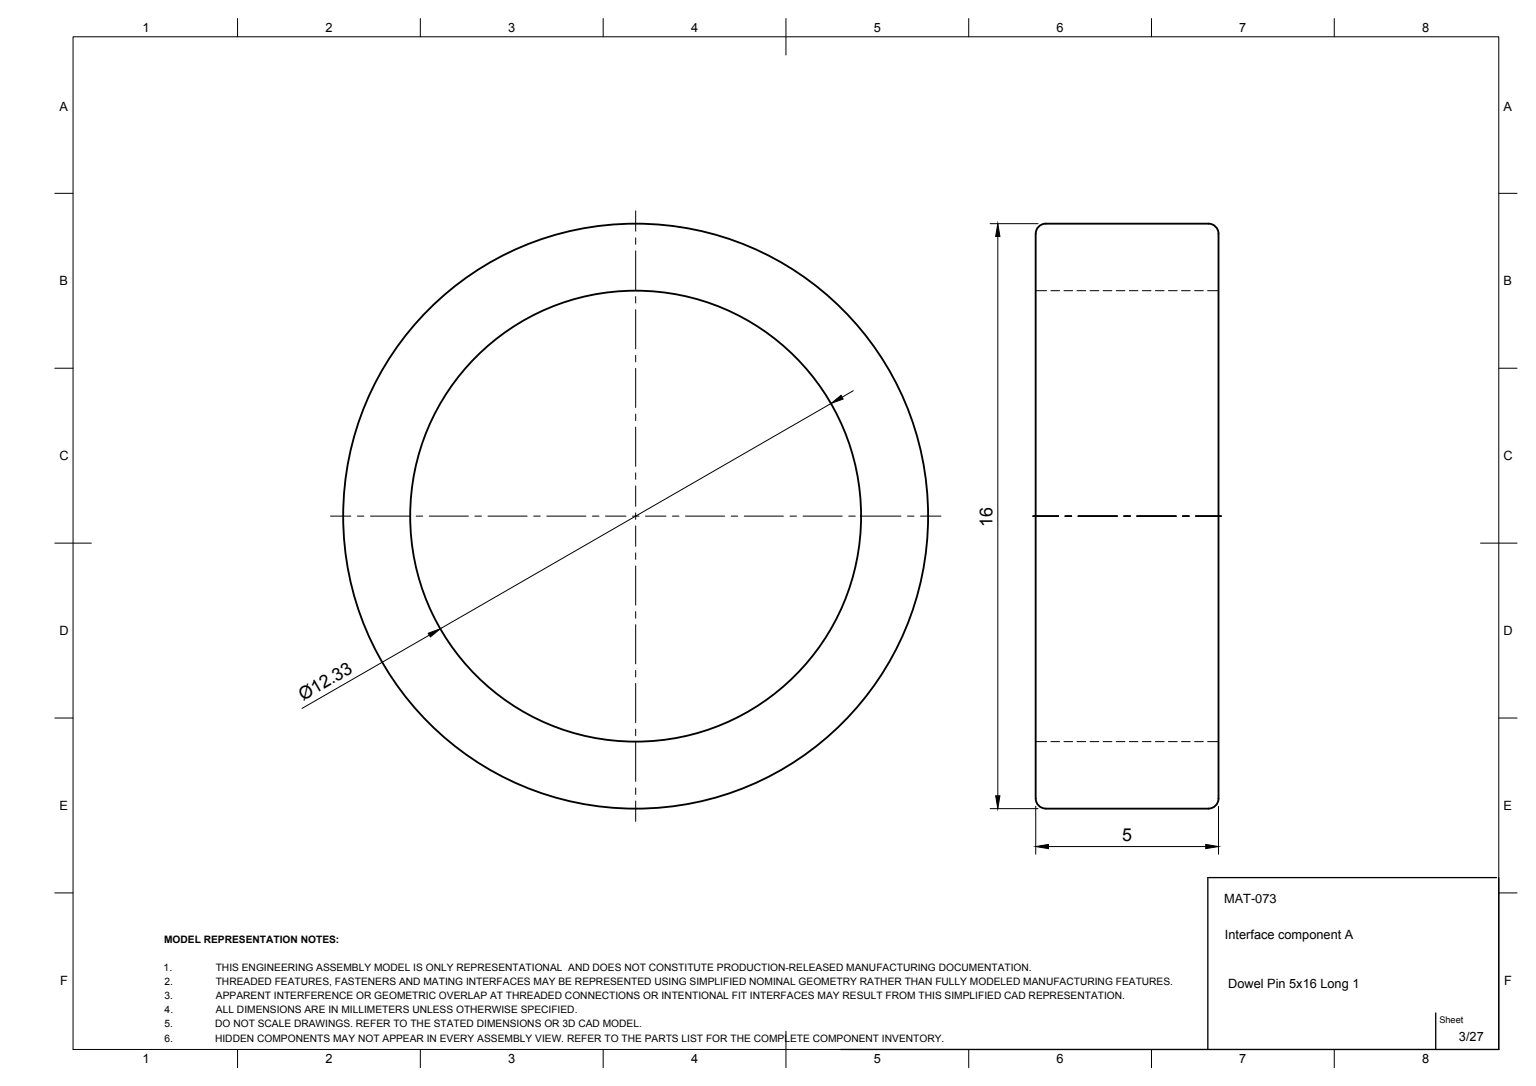
ISO-10303-21;
HEADER;
/* Generated by software containing ST-Developer
 * from STEP Tools, Inc. (www.steptools.com) 
 */

FILE_DESCRIPTION(
/* description */ ('CAx-IF Rec.Pracs.---Representation and Presentation of Product Manufa
cturing Information (PMI)---4.0---2014-10-13'),
/* implementation_level */ '2;1');

FILE_NAME(
/* name */ 'Interface component A.step',
/* time_stamp */ '2026-10-24T18:52:33-07:00',
/* author */ (''),
/* organization */ (''),
/* preprocessor_version */ 'ST-DEVELOPER v20.2',
/* originating_system */ 'Autodesk Translation Framework v15.17.0.0',
/* authorisation */ '');

FILE_SCHEMA (('AP242_MANAGED_MODEL_BASED_3D_ENGINEERING_MIM_LF { 1 0 10303 442 2 1 4 }'));
ENDSEC;

DATA;
#10=MECHANICAL_DESIGN_GEOMETRIC_PRESENTATION_REPRESENTATION('',(#414),#34876);
#348=SHAPE_REPRESENTATION_RELATIONSHIP('SRR','None',#34985,#381);
#381=ADVANCED_BREP_SHAPE_REPRESENTATION('',(#447),#34843);
#414=STYLED_ITEM('',(#35159),#447);
#447=MANIFOLD_SOLID_BREP('Dowel Pin 5x16 Long 1',#19554);
#480=FACE_BOUND('',#5841,.T.);
#481=FACE_BOUND('',#5844,.T.);
#590=PLANE('',#19961);
#591=PLANE('',#19966);
#1083=LINE('',#28483,#2682);
#1084=LINE('',#28498,#2683);
#2682=VECTOR('',#22274,0.008);
#2683=VECTOR('',#22295,0.00616666666666666);
#4281=CYLINDRICAL_SURFACE('',#19958,0.008);
#4282=CYLINDRICAL_SURFACE('',#19968,0.00616666666666666);
#4793=FACE_OUTER_BOUND('',#5838,.T.);
#4794=FACE_OUTER_BOUND('',#5839,.T.);
#4795=FACE_OUTER_BOUND('',#5840,.T.);
#4796=FACE_OUTER_BOUND('',#5842,.T.);
#4797=FACE_OUTER_BOUND('',#5843,.T.);
#4798=FACE_OUTER_BOUND('',#5845,.T.);
#5838=EDGE_LOOP('',(#12806,#12807,#12808,#12809,#12810));
#5839=EDGE_LOOP('',(#12811,#12812,#12813,#12814,#12815,#12816));
#5840=EDGE_LOOP('',(#12817));
#5841=EDGE_LOOP('',(#12818));
#5842=EDGE_LOOP('',(#12819,#12820,#12821,#12822,#12823));
#5843=EDGE_LOOP('',(#12824));
#5844=EDGE_LOOP('',(#12825));
#5845=EDGE_LOOP('',(#12826,#12827,#12828,#12829));
#6993=CIRCLE('',#19954,0.00772500000001);
#6994=CIRCLE('',#19955,0.000275);
#6995=CIRCLE('',#19956,0.00800000000001);
#6996=CIRCLE('',#19957,0.00800000000001);
#6997=CIRCLE('',#19959,0.00800000000001);
#6998=CIRCLE('',#19960,0.00800000000001);
#6999=CIRCLE('',#19962,0.00616666666667666);
#7000=CIRCLE('',#19964,0.000275);
#7001=CIRCLE('',#19965,0.00772500000001);
#7002=CIRCLE('',#19967,0.00616666666667666);
#8073=VERTEX_POINT('',#28474);
#8074=VERTEX_POINT('',#28476);
#8075=VERTEX_POINT('',#28478);
#8076=VERTEX_POINT('',#28482);
#8077=VERTEX_POINT('',#28484);
#8078=VERTEX_POINT('',#28488);
#8079=VERTEX_POINT('',#28491);
#8080=VERTEX_POINT('',#28495);
#9961=EDGE_CURVE('',#8073,#8073,#6993,.T.);
#9962=EDGE_CURVE('',#8073,#8074,#6994,.T.);
#9963=EDGE_CURVE('',#8074,#8075,#6995,.T.);
#9964=EDGE_CURVE('',#8075,#8074,#6996,.T.);
#9965=EDGE_CURVE('',#8075,#8076,#1083,.T.);
#9966=EDGE_CURVE('',#8077,#8076,#6997,.T.);
#9967=EDGE_CURVE('',#8076,#8077,#6998,.T.);
#9968=EDGE_CURVE('',#8078,#8078,#6999,.T.);
#9969=EDGE_CURVE('',#8077,#8079,#7000,.T.);
#9970=EDGE_CURVE('',#8079,#8079,#7001,.T.);
#9971=EDGE_CURVE('',#8080,#8080,#7002,.T.);
#9972=EDGE_CURVE('',#8080,#8078,#1084,.T.);
#12806=ORIENTED_EDGE('',*,*,#9961,.T.);
#12807=ORIENTED_EDGE('',*,*,#9962,.T.);
#12808=ORIENTED_EDGE('',*,*,#9963,.T.);
#12809=ORIENTED_EDGE('',*,*,#9964,.T.);
#12810=ORIENTED_EDGE('',*,*,#9962,.F.);
#12811=ORIENTED_EDGE('',*,*,#9964,.F.);
#12812=ORIENTED_EDGE('',*,*,#9965,.T.);
#12813=ORIENTED_EDGE('',*,*,#9966,.F.);
#12814=ORIENTED_EDGE('',*,*,#9967,.F.);
#12815=ORIENTED_EDGE('',*,*,#9965,.F.);
#12816=ORIENTED_EDGE('',*,*,#9963,.F.);
#12817=ORIENTED_EDGE('',*,*,#9961,.F.);
#12818=ORIENTED_EDGE('',*,*,#9968,.F.);
#12819=ORIENTED_EDGE('',*,*,#9967,.T.);
#12820=ORIENTED_EDGE('',*,*,#9969,.T.);
#12821=ORIENTED_EDGE('',*,*,#9970,.T.);
#12822=ORIENTED_EDGE('',*,*,#9969,.F.);
#12823=ORIENTED_EDGE('',*,*,#9966,.T.);
#12824=ORIENTED_EDGE('',*,*,#9970,.F.);
#12825=ORIENTED_EDGE('',*,*,#9971,.T.);
#12826=ORIENTED_EDGE('',*,*,#9971,.F.);
#12827=ORIENTED_EDGE('',*,*,#9972,.T.);
#12828=ORIENTED_EDGE('',*,*,#9968,.T.);
#12829=ORIENTED_EDGE('',*,*,#9972,.F.);
#18496=TOROIDAL_SURFACE('',#19953,0.007725,0.000275);
#18497=TOROIDAL_SURFACE('',#19963,0.007725,0.000275);
#18509=ADVANCED_FACE('',(#4793),#18496,.T.);
#18510=ADVANCED_FACE('',(#4794),#4281,.T.);
#18511=ADVANCED_FACE('',(#4795,#480),#590,.T.);
#18512=ADVANCED_FACE('',(#4796),#18497,.T.);
#18513=ADVANCED_FACE('',(#4797,#481),#591,.T.);
#18514=ADVANCED_FACE('',(#4798),#4282,.F.);
#19554=CLOSED_SHELL('',(#18509,#18510,#18511,#18512,#18513,#18514));
#19952=AXIS2_PLACEMENT_3D('',#28472,#22260,#22261);
#19953=AXIS2_PLACEMENT_3D('',#28473,#22262,#22263);
#19954=AXIS2_PLACEMENT_3D('',#28475,#22264,#22265);
#19955=AXIS2_PLACEMENT_3D('',#28477,#22266,#22267);
#19956=AXIS2_PLACEMENT_3D('',#28479,#22268,#22269);
#19957=AXIS2_PLACEMENT_3D('',#28480,#22270,#22271);
#19958=AXIS2_PLACEMENT_3D('',#28481,#22272,#22273);
#19959=AXIS2_PLACEMENT_3D('',#28485,#22275,#22276);
#19960=AXIS2_PLACEMENT_3D('',#28486,#22277,#22278);
#19961=AXIS2_PLACEMENT_3D('',#28487,#22279,#22280);
#19962=AXIS2_PLACEMENT_3D('',#28489,#22281,#22282);
#19963=AXIS2_PLACEMENT_3D('',#28490,#22283,#22284);
#19964=AXIS2_PLACEMENT_3D('',#28492,#22285,#22286);
#19965=AXIS2_PLACEMENT_3D('',#28493,#22287,#22288);
#19966=AXIS2_PLACEMENT_3D('',#28494,#22289,#22290);
#19967=AXIS2_PLACEMENT_3D('',#28496,#22291,#22292);
#19968=AXIS2_PLACEMENT_3D('',#28497,#22293,#22294);
#22260=DIRECTION('axis',(0.,0.,1.));
#22261=DIRECTION('refdir',(1.,0.,0.));
#22262=DIRECTION('center_axis',(4.55032717710333E-17,-1.,1.51850909121962E-32));
#22263=DIRECTION('ref_axis',(-0.770184521566975,0.,0.637821136948792));
#22264=DIRECTION('center_axis',(-4.55032717710333E-17,1.,-1.51850909121962E-32));
#22265=DIRECTION('ref_axis',(0.637821136949789,2.90229485359357E-17,0.770184521566149));
#22266=DIRECTION('center_axis',(0.637821136948792,2.90229485358903E-17,
0.770184521566975));
#22267=DIRECTION('ref_axis',(0.770184521566975,0.,-0.637821136948792));
#22268=DIRECTION('center_axis',(4.55032717710333E-17,-1.,1.51850909121962E-32));
#22269=DIRECTION('ref_axis',(0.637821136949755,2.90229485359342E-17,0.770184521566178));
#22270=DIRECTION('center_axis',(4.55032717710333E-17,-1.,1.51850909121962E-32));
#22271=DIRECTION('ref_axis',(0.637821136949755,2.90229485359342E-17,0.770184521566178));
#22272=DIRECTION('center_axis',(4.55032717710333E-17,-1.,1.51850909121962E-32));
#22273=DIRECTION('ref_axis',(-0.637821136948792,-2.90229485358903E-17,-0.770184521566975));
#22274=DIRECTION('',(-4.55032717710333E-17,1.,-1.51850909121962E-32));
#22275=DIRECTION('center_axis',(-4.55032717710333E-17,1.,-1.51850909121962E-32));
#22276=DIRECTION('ref_axis',(0.637821136949755,2.90229485359342E-17,0.770184521566178));
#22277=DIRECTION('center_axis',(-4.55032717710333E-17,1.,-1.51850909121962E-32));
#22278=DIRECTION('ref_axis',(0.637821136949755,2.90229485359342E-17,0.770184521566178));
#22279=DIRECTION('center_axis',(4.55032717710333E-17,-1.,1.51850909121962E-32));
#22280=DIRECTION('ref_axis',(-0.637821136948792,-2.90229485358903E-17,-0.770184521566975));
#22281=DIRECTION('center_axis',(4.55032717710333E-17,-1.,1.51850909121962E-32));
#22282=DIRECTION('ref_axis',(-0.637821136948792,-2.90229485358904E-17,-0.770184521566975));
#22283=DIRECTION('center_axis',(4.55032717710333E-17,-1.,1.51850909121962E-32));
#22284=DIRECTION('ref_axis',(-0.770184521566975,-5.42101086242752E-17,0.637821136948792));
#22285=DIRECTION('center_axis',(0.637821136948792,2.90229485358903E-17,
0.770184521566975));
#22286=DIRECTION('ref_axis',(0.770184521566975,3.46944695195361E-17,-0.637821136948792));
#22287=DIRECTION('center_axis',(4.55032717710333E-17,-1.,1.51850909121962E-32));
#22288=DIRECTION('ref_axis',(0.637821136949789,2.90229485359357E-17,0.770184521566149));
#22289=DIRECTION('center_axis',(-4.55032717710333E-17,1.,-1.51850909121962E-32));
#22290=DIRECTION('ref_axis',(0.770184521566975,3.50459155987053E-17,-0.637821136948792));
#22291=DIRECTION('center_axis',(4.55032717710333E-17,-1.,1.51850909121962E-32));
#22292=DIRECTION('ref_axis',(-0.637821136948792,-2.90229485358904E-17,-0.770184521566975));
#22293=DIRECTION('center_axis',(4.55032717710333E-17,-1.,1.51850909121962E-32));
#22294=DIRECTION('ref_axis',(-0.637821136948792,-2.90229485358903E-17,-0.770184521566975));
#22295=DIRECTION('',(4.55032717710333E-17,-1.,1.51850909121962E-32));
#28472=CARTESIAN_POINT('',(0.,0.,0.));
#28473=CARTESIAN_POINT('Origin',(-4.50826289289608E-17,-0.006725,1.13636778952413E-32));
#28474=CARTESIAN_POINT('',(0.00594967542911254,-0.00700000000001,-0.00492716828293579));
#28475=CARTESIAN_POINT('Origin',(-4.50701155292233E-17,-0.00700000000001,
1.13678537952423E-32));
#28476=CARTESIAN_POINT('',(0.00616147617254346,-0.00672500000001,-0.00510256909559671));
#28477=CARTESIAN_POINT('Origin',(0.00594967542910484,-0.006725,-0.00492716828292942));
#28478=CARTESIAN_POINT('',(0.00510256909560437,-0.00672500000001,0.00616147617253713));
#28479=CARTESIAN_POINT('Origin',(-4.50826289289603E-17,-0.00672500000001,
1.13636778952415E-32));
#28480=CARTESIAN_POINT('Origin',(-4.50826289289603E-17,-0.00672500000001,
1.13636778952415E-32));
#28481=CARTESIAN_POINT('Origin',(-4.51838737086513E-17,-0.0045,1.13298910679617E-32));
#28482=CARTESIAN_POINT('',(0.00510256909560437,-0.00227500000001,0.00616147617253713));
#28483=CARTESIAN_POINT('',(0.00510256909559029,-0.0045,0.0061614761725358));
#28484=CARTESIAN_POINT('',(0.00616147617254346,-0.00227500000001001,-0.00510256909559671));
#28485=CARTESIAN_POINT('Origin',(-4.52851184883414E-17,-0.00227500000001001,
1.12961042406822E-32));
#28486=CARTESIAN_POINT('Origin',(-4.52851184883414E-17,-0.00227500000001001,
1.12961042406822E-32));
#28487=CARTESIAN_POINT('Origin',(-0.00451789972005399,-0.007,-0.00545547369443274));
#28488=CARTESIAN_POINT('',(0.0039332303445175,-0.00700000000001,0.00474947121632968));
#28489=CARTESIAN_POINT('Origin',(-4.50701155292233E-17,-0.00700000000001,
1.13678537952423E-32));
#28490=CARTESIAN_POINT('Origin',(-4.52851184883419E-17,-0.002275,1.1296104240682E-32));
#28491=CARTESIAN_POINT('',(0.00594967542911254,-0.00200000000001001,-0.00492716828293579));
#28492=CARTESIAN_POINT('Origin',(0.00594967542910484,-0.002275,-0.00492716828292942));
#28493=CARTESIAN_POINT('Origin',(-4.52976318880785E-17,-0.00200000000001001,
1.12919283406813E-32));
#28494=CARTESIAN_POINT('Origin',(-0.00451789972005399,-0.002,-0.00545547369443274));
#28495=CARTESIAN_POINT('',(0.0039332303445175,-0.00200000000001001,0.00474947121632968));
#28496=CARTESIAN_POINT('Origin',(-4.52976318880785E-17,-0.00200000000001001,
1.12919283406813E-32));
#28497=CARTESIAN_POINT('Origin',(-4.51838737086513E-17,-0.0045,1.13298910679617E-32));
#28498=CARTESIAN_POINT('',(0.0039332303445175,-0.0045,0.00474947121632968));
#34808=UNCERTAINTY_MEASURE_WITH_UNIT(LENGTH_MEASURE(1.E-5),#34877,
'DISTANCE_ACCURACY_VALUE',
'Maximum model space distance between geometric entities at asserted c
onnectivities');
#34841=UNCERTAINTY_MEASURE_WITH_UNIT(LENGTH_MEASURE(1.E-5),#34877,
'DISTANCE_ACCURACY_VALUE',
'Maximum model space distance between geometric entities at asserted c
onnectivities');
#34843=(
GEOMETRIC_REPRESENTATION_CONTEXT(3)
GLOBAL_UNCERTAINTY_ASSIGNED_CONTEXT((#34808))
GLOBAL_UNIT_ASSIGNED_CONTEXT((#34877,#34878,#34879))
REPRESENTATION_CONTEXT('','3D')
);
#34876=(
GEOMETRIC_REPRESENTATION_CONTEXT(3)
GLOBAL_UNCERTAINTY_ASSIGNED_CONTEXT((#34841))
GLOBAL_UNIT_ASSIGNED_CONTEXT((#34877,#34878,#34879))
REPRESENTATION_CONTEXT('','3D')
);
#34877=(
LENGTH_UNIT()
NAMED_UNIT(*)
SI_UNIT($,.METRE.)
);
#34878=(
NAMED_UNIT(*)
PLANE_ANGLE_UNIT()
SI_UNIT($,.RADIAN.)
);
#34879=(
NAMED_UNIT(*)
SI_UNIT($,.STERADIAN.)
SOLID_ANGLE_UNIT()
);
#34881=SHAPE_DEFINITION_REPRESENTATION(#34915,#34985);
#34915=PRODUCT_DEFINITION_SHAPE('',$,#35020);
#34985=SHAPE_REPRESENTATION('',(#19952),#34843);
#35018=PRODUCT_DEFINITION_CONTEXT('part definition',#35122,'design');
#35020=PRODUCT_DEFINITION('Interface component A',
'Interface component A',#35054,#35018);
#35054=PRODUCT_DEFINITION_FORMATION('',$,#35125);
#35122=APPLICATION_CONTEXT('Managed model based 3d engineering');
#35123=PRODUCT_CONTEXT('part definition',#35122,'mechanical');
#35125=PRODUCT('Interface component A','Interface component A',
'LEGAL AND USAGE DISCLAIMER: this Data/Model is provided \X2\201C\X0\A
S IS\X2\201D\X0\ for informational and representational only. It is a 
geometric approximation and is NOT engineered, certified, or guarantee
d for dimensional accuracy, exact tolerances, or production-level prec
ision. Vendor disclaims all implied warranties including fitness for a
 particular purpose. DO NOT USE FOR DIRECT PHYSICAL MANUFACTURING, AUT
OMATED PRODUCTION, OR SAFETY-CRITICAL SYSTEMS without independent engi
neering verification and resolution of any design discrepancies.',(#35123));
#35159=PRESENTATION_STYLE_ASSIGNMENT((#35168));
#35168=SURFACE_STYLE_USAGE(.BOTH.,#35177);
#35177=SURFACE_SIDE_STYLE('',(#35186));
#35186=SURFACE_STYLE_FILL_AREA(#35195);
#35195=FILL_AREA_STYLE('Paint - Enamel Glossy (White)',(#35204));
#35204=FILL_AREA_STYLE_COLOUR('Paint - Enamel Glossy (White)',#35213);
#35213=COLOUR_RGB('Paint - Enamel Glossy (White)',0.964705882352941,0.964705882352941,
0.952941176470588);
ENDSEC;
END-ISO-10303-21;
